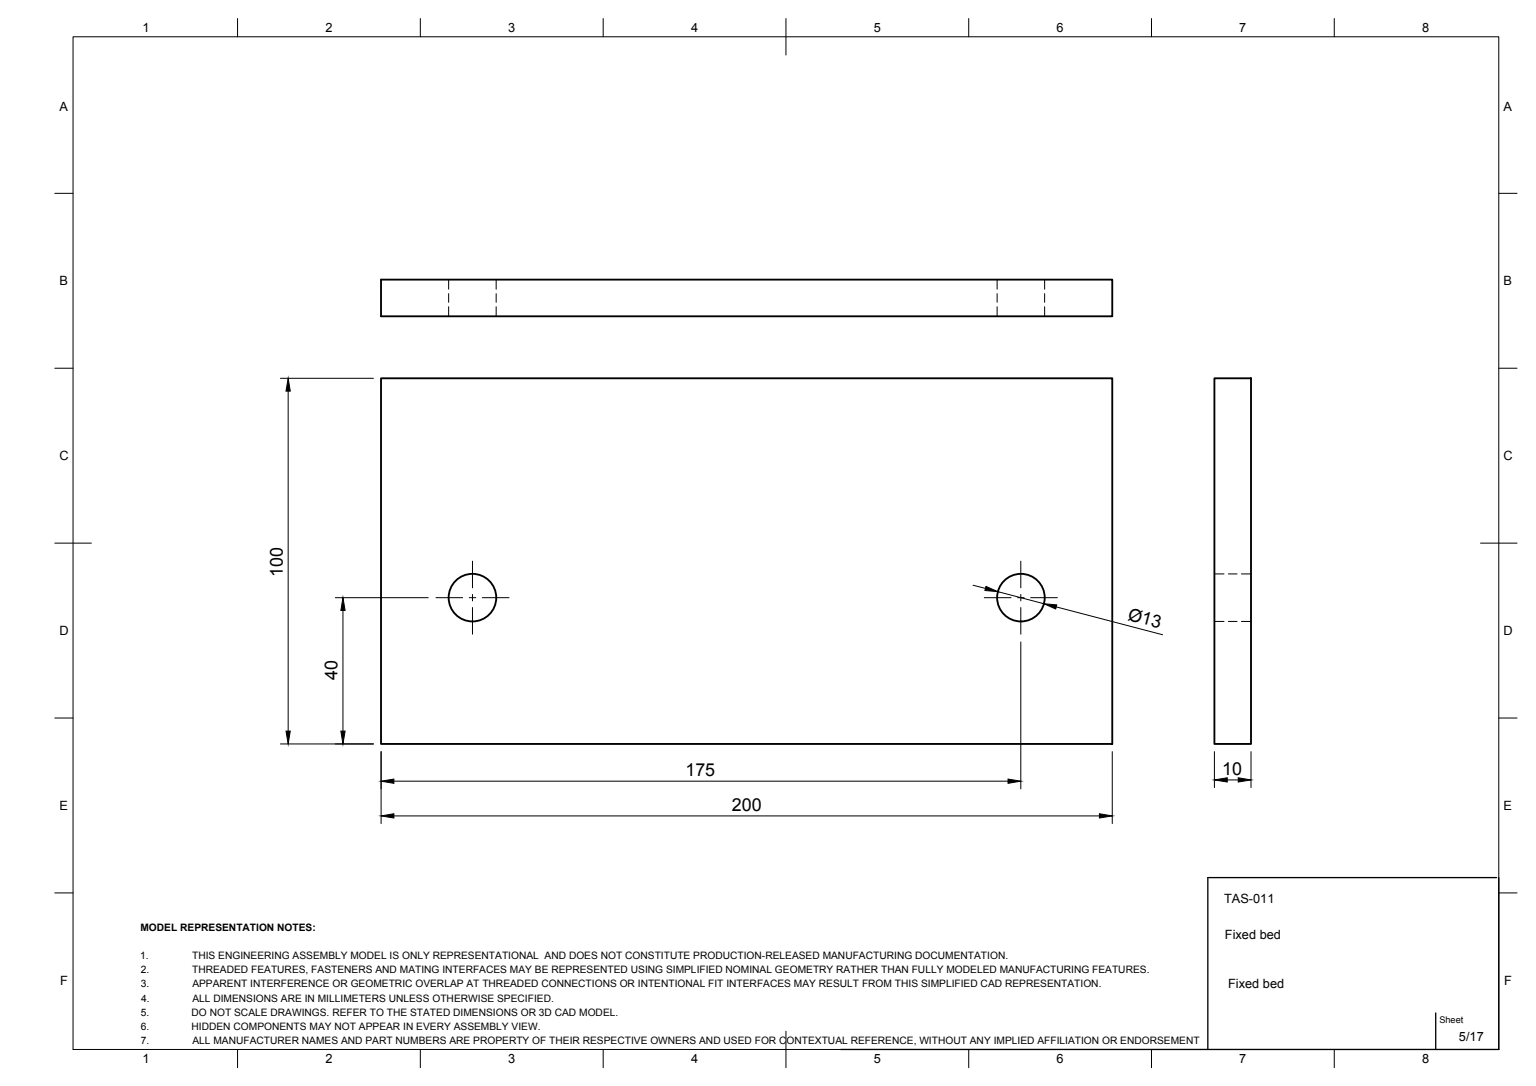
ISO-10303-21;
HEADER;
/* Generated by software containing ST-Developer
 * from STEP Tools, Inc. (www.steptools.com) 
 */

FILE_DESCRIPTION(
/* description */ (
'Independent manual bench leaf bending machine,200mm work width. Fabri
cated welded frame and folding leaf, repeated bushed and fully retaine
d hinge hardware, two handles with bonded grips, beveled clamping beam
 and modeledM12 clamp screws.2mm omitted-workpiece assembly reference 
gap, not a capacity claim. Native135deg hinge travel. Weld sizing, pro
duction fits, material condition, bending capacity, strength and life 
unassigned.'),
/* implementation_level */ '2;1');

FILE_NAME(
/* name */ 'Fixed bed.step',
/* time_stamp */ '2026-11-14T09:11:34-08:00',
/* author */ (''),
/* organization */ (''),
/* preprocessor_version */ 'ST-DEVELOPER v20.2',
/* originating_system */ 'Autodesk Translation Framework v15.17.0.0',
/* authorisation */ '');

FILE_SCHEMA (('AUTOMOTIVE_DESIGN { 1 0 10303 214 3 1 1 }'));
ENDSEC;

DATA;
#10=MECHANICAL_DESIGN_GEOMETRIC_PRESENTATION_REPRESENTATION('',(#447),#37701);
#411=SHAPE_REPRESENTATION_RELATIONSHIP('SRR','None',#37780,#429);
#429=ADVANCED_BREP_SHAPE_REPRESENTATION('',(#465),#37684);
#447=STYLED_ITEM('',(#37879),#465);
#465=MANIFOLD_SOLID_BREP('Body1',#4145);
#490=FACE_BOUND('',#843,.T.);
#491=FACE_BOUND('',#844,.T.);
#492=FACE_BOUND('',#846,.T.);
#493=FACE_BOUND('',#847,.T.);
#522=PLANE('',#4400);
#523=PLANE('',#4401);
#524=PLANE('',#4402);
#525=PLANE('',#4403);
#526=PLANE('',#4404);
#527=PLANE('',#4405);
#616=FACE_OUTER_BOUND('',#836,.T.);
#617=FACE_OUTER_BOUND('',#837,.T.);
#618=FACE_OUTER_BOUND('',#838,.T.);
#619=FACE_OUTER_BOUND('',#839,.T.);
#620=FACE_OUTER_BOUND('',#840,.T.);
#621=FACE_OUTER_BOUND('',#841,.T.);
#622=FACE_OUTER_BOUND('',#842,.T.);
#623=FACE_OUTER_BOUND('',#845,.T.);
#836=EDGE_LOOP('',(#2711,#2712,#2713,#2714));
#837=EDGE_LOOP('',(#2715,#2716,#2717,#2718));
#838=EDGE_LOOP('',(#2719,#2720,#2721,#2722));
#839=EDGE_LOOP('',(#2723,#2724,#2725,#2726));
#840=EDGE_LOOP('',(#2727,#2728,#2729,#2730));
#841=EDGE_LOOP('',(#2731,#2732,#2733,#2734));
#842=EDGE_LOOP('',(#2735,#2736,#2737,#2738));
#843=EDGE_LOOP('',(#2739));
#844=EDGE_LOOP('',(#2740));
#845=EDGE_LOOP('',(#2741,#2742,#2743,#2744));
#846=EDGE_LOOP('',(#2745));
#847=EDGE_LOOP('',(#2746));
#1080=LINE('',#5729,#1329);
#1081=LINE('',#5735,#1330);
#1082=LINE('',#5740,#1331);
#1083=LINE('',#5742,#1332);
#1084=LINE('',#5744,#1333);
#1085=LINE('',#5745,#1334);
#1086=LINE('',#5748,#1335);
#1087=LINE('',#5750,#1336);
#1088=LINE('',#5751,#1337);
#1089=LINE('',#5754,#1338);
#1090=LINE('',#5756,#1339);
#1091=LINE('',#5757,#1340);
#1092=LINE('',#5759,#1341);
#1093=LINE('',#5760,#1342);
#1329=VECTOR('',#4797,6.5);
#1330=VECTOR('',#4804,6.5);
#1331=VECTOR('',#4809,10.);
#1332=VECTOR('',#4810,10.);
#1333=VECTOR('',#4811,10.);
#1334=VECTOR('',#4812,10.);
#1335=VECTOR('',#4815,10.);
#1336=VECTOR('',#4816,10.);
#1337=VECTOR('',#4817,10.);
#1338=VECTOR('',#4820,10.);
#1339=VECTOR('',#4821,10.);
#1340=VECTOR('',#4822,10.);
#1341=VECTOR('',#4825,10.);
#1342=VECTOR('',#4826,10.);
#1574=CIRCLE('',#4395,6.5);
#1575=CIRCLE('',#4396,6.5);
#1576=CIRCLE('',#4398,6.5);
#1577=CIRCLE('',#4399,6.5);
#1661=VERTEX_POINT('',#5726);
#1662=VERTEX_POINT('',#5728);
#1663=VERTEX_POINT('',#5732);
#1664=VERTEX_POINT('',#5734);
#1665=VERTEX_POINT('',#5738);
#1666=VERTEX_POINT('',#5739);
#1667=VERTEX_POINT('',#5741);
#1668=VERTEX_POINT('',#5743);
#1669=VERTEX_POINT('',#5747);
#1670=VERTEX_POINT('',#5749);
#1671=VERTEX_POINT('',#5753);
#1672=VERTEX_POINT('',#5755);
#2089=EDGE_CURVE('',#1661,#1661,#1574,.T.);
#2090=EDGE_CURVE('',#1661,#1662,#1080,.T.);
#2091=EDGE_CURVE('',#1662,#1662,#1575,.T.);
#2092=EDGE_CURVE('',#1663,#1663,#1576,.T.);
#2093=EDGE_CURVE('',#1663,#1664,#1081,.T.);
#2094=EDGE_CURVE('',#1664,#1664,#1577,.T.);
#2095=EDGE_CURVE('',#1665,#1666,#1082,.T.);
#2096=EDGE_CURVE('',#1666,#1667,#1083,.T.);
#2097=EDGE_CURVE('',#1668,#1667,#1084,.T.);
#2098=EDGE_CURVE('',#1665,#1668,#1085,.T.);
#2099=EDGE_CURVE('',#1669,#1665,#1086,.T.);
#2100=EDGE_CURVE('',#1670,#1668,#1087,.T.);
#2101=EDGE_CURVE('',#1669,#1670,#1088,.T.);
#2102=EDGE_CURVE('',#1671,#1669,#1089,.T.);
#2103=EDGE_CURVE('',#1672,#1670,#1090,.T.);
#2104=EDGE_CURVE('',#1671,#1672,#1091,.T.);
#2105=EDGE_CURVE('',#1666,#1671,#1092,.T.);
#2106=EDGE_CURVE('',#1667,#1672,#1093,.T.);
#2711=ORIENTED_EDGE('',*,*,#2089,.F.);
#2712=ORIENTED_EDGE('',*,*,#2090,.T.);
#2713=ORIENTED_EDGE('',*,*,#2091,.F.);
#2714=ORIENTED_EDGE('',*,*,#2090,.F.);
#2715=ORIENTED_EDGE('',*,*,#2092,.F.);
#2716=ORIENTED_EDGE('',*,*,#2093,.T.);
#2717=ORIENTED_EDGE('',*,*,#2094,.F.);
#2718=ORIENTED_EDGE('',*,*,#2093,.F.);
#2719=ORIENTED_EDGE('',*,*,#2095,.T.);
#2720=ORIENTED_EDGE('',*,*,#2096,.T.);
#2721=ORIENTED_EDGE('',*,*,#2097,.F.);
#2722=ORIENTED_EDGE('',*,*,#2098,.F.);
#2723=ORIENTED_EDGE('',*,*,#2099,.T.);
#2724=ORIENTED_EDGE('',*,*,#2098,.T.);
#2725=ORIENTED_EDGE('',*,*,#2100,.F.);
#2726=ORIENTED_EDGE('',*,*,#2101,.F.);
#2727=ORIENTED_EDGE('',*,*,#2102,.T.);
#2728=ORIENTED_EDGE('',*,*,#2101,.T.);
#2729=ORIENTED_EDGE('',*,*,#2103,.F.);
#2730=ORIENTED_EDGE('',*,*,#2104,.F.);
#2731=ORIENTED_EDGE('',*,*,#2105,.T.);
#2732=ORIENTED_EDGE('',*,*,#2104,.T.);
#2733=ORIENTED_EDGE('',*,*,#2106,.F.);
#2734=ORIENTED_EDGE('',*,*,#2096,.F.);
#2735=ORIENTED_EDGE('',*,*,#2106,.T.);
#2736=ORIENTED_EDGE('',*,*,#2103,.T.);
#2737=ORIENTED_EDGE('',*,*,#2100,.T.);
#2738=ORIENTED_EDGE('',*,*,#2097,.T.);
#2739=ORIENTED_EDGE('',*,*,#2089,.T.);
#2740=ORIENTED_EDGE('',*,*,#2092,.T.);
#2741=ORIENTED_EDGE('',*,*,#2105,.F.);
#2742=ORIENTED_EDGE('',*,*,#2095,.F.);
#2743=ORIENTED_EDGE('',*,*,#2099,.F.);
#2744=ORIENTED_EDGE('',*,*,#2102,.F.);
#2745=ORIENTED_EDGE('',*,*,#2091,.T.);
#2746=ORIENTED_EDGE('',*,*,#2094,.T.);
#3819=CYLINDRICAL_SURFACE('',#4394,6.5);
#3820=CYLINDRICAL_SURFACE('',#4397,6.5);
#3946=ADVANCED_FACE('',(#616),#3819,.F.);
#3947=ADVANCED_FACE('',(#617),#3820,.F.);
#3948=ADVANCED_FACE('',(#618),#522,.T.);
#3949=ADVANCED_FACE('',(#619),#523,.T.);
#3950=ADVANCED_FACE('',(#620),#524,.T.);
#3951=ADVANCED_FACE('',(#621),#525,.T.);
#3952=ADVANCED_FACE('',(#622,#490,#491),#526,.T.);
#3953=ADVANCED_FACE('',(#623,#492,#493),#527,.F.);
#4145=CLOSED_SHELL('',(#3946,#3947,#3948,#3949,#3950,#3951,#3952,#3953));
#4393=AXIS2_PLACEMENT_3D('',#5724,#4791,#4792);
#4394=AXIS2_PLACEMENT_3D('',#5725,#4793,#4794);
#4395=AXIS2_PLACEMENT_3D('',#5727,#4795,#4796);
#4396=AXIS2_PLACEMENT_3D('',#5730,#4798,#4799);
#4397=AXIS2_PLACEMENT_3D('',#5731,#4800,#4801);
#4398=AXIS2_PLACEMENT_3D('',#5733,#4802,#4803);
#4399=AXIS2_PLACEMENT_3D('',#5736,#4805,#4806);
#4400=AXIS2_PLACEMENT_3D('',#5737,#4807,#4808);
#4401=AXIS2_PLACEMENT_3D('',#5746,#4813,#4814);
#4402=AXIS2_PLACEMENT_3D('',#5752,#4818,#4819);
#4403=AXIS2_PLACEMENT_3D('',#5758,#4823,#4824);
#4404=AXIS2_PLACEMENT_3D('',#5761,#4827,#4828);
#4405=AXIS2_PLACEMENT_3D('',#5762,#4829,#4830);
#4791=DIRECTION('axis',(0.,0.,1.));
#4792=DIRECTION('refdir',(1.,0.,0.));
#4793=DIRECTION('center_axis',(0.,0.,-1.));
#4794=DIRECTION('ref_axis',(1.,0.,0.));
#4795=DIRECTION('center_axis',(0.,0.,-1.));
#4796=DIRECTION('ref_axis',(1.,0.,0.));
#4797=DIRECTION('',(0.,0.,-1.));
#4798=DIRECTION('center_axis',(0.,0.,1.));
#4799=DIRECTION('ref_axis',(1.,0.,0.));
#4800=DIRECTION('center_axis',(0.,0.,-1.));
#4801=DIRECTION('ref_axis',(1.,0.,0.));
#4802=DIRECTION('center_axis',(0.,0.,-1.));
#4803=DIRECTION('ref_axis',(1.,0.,0.));
#4804=DIRECTION('',(0.,0.,-1.));
#4805=DIRECTION('center_axis',(0.,0.,1.));
#4806=DIRECTION('ref_axis',(1.,0.,0.));
#4807=DIRECTION('center_axis',(0.,1.,0.));
#4808=DIRECTION('ref_axis',(-1.,0.,0.));
#4809=DIRECTION('',(-1.,0.,0.));
#4810=DIRECTION('',(0.,0.,1.));
#4811=DIRECTION('',(-1.,0.,0.));
#4812=DIRECTION('',(0.,0.,1.));
#4813=DIRECTION('center_axis',(1.,0.,0.));
#4814=DIRECTION('ref_axis',(0.,1.,0.));
#4815=DIRECTION('',(0.,1.,0.));
#4816=DIRECTION('',(0.,1.,0.));
#4817=DIRECTION('',(0.,0.,1.));
#4818=DIRECTION('center_axis',(0.,-1.,0.));
#4819=DIRECTION('ref_axis',(1.,0.,0.));
#4820=DIRECTION('',(1.,0.,0.));
#4821=DIRECTION('',(1.,0.,0.));
#4822=DIRECTION('',(0.,0.,1.));
#4823=DIRECTION('center_axis',(-1.,0.,0.));
#4824=DIRECTION('ref_axis',(0.,-1.,0.));
#4825=DIRECTION('',(0.,-1.,0.));
#4826=DIRECTION('',(0.,-1.,0.));
#4827=DIRECTION('center_axis',(0.,0.,1.));
#4828=DIRECTION('ref_axis',(1.,0.,0.));
#4829=DIRECTION('center_axis',(0.,0.,1.));
#4830=DIRECTION('ref_axis',(1.,0.,0.));
#5724=CARTESIAN_POINT('',(0.,0.,0.));
#5725=CARTESIAN_POINT('Origin',(-60.,-75.,35.));
#5726=CARTESIAN_POINT('',(-66.5,-75.,40.));
#5727=CARTESIAN_POINT('Origin',(-60.,-75.,40.));
#5728=CARTESIAN_POINT('',(-66.5,-75.,30.));
#5729=CARTESIAN_POINT('',(-66.5,-75.,35.));
#5730=CARTESIAN_POINT('Origin',(-60.,-75.,30.));
#5731=CARTESIAN_POINT('Origin',(-60.,75.,35.));
#5732=CARTESIAN_POINT('',(-66.5,75.,40.));
#5733=CARTESIAN_POINT('Origin',(-60.,75.,40.));
#5734=CARTESIAN_POINT('',(-66.5,75.,30.));
#5735=CARTESIAN_POINT('',(-66.5,75.,35.));
#5736=CARTESIAN_POINT('Origin',(-60.,75.,30.));
#5737=CARTESIAN_POINT('Origin',(0.,100.,30.));
#5738=CARTESIAN_POINT('',(0.,100.,30.));
#5739=CARTESIAN_POINT('',(-100.,100.,30.));
#5740=CARTESIAN_POINT('',(0.,100.,30.));
#5741=CARTESIAN_POINT('',(-100.,100.,40.));
#5742=CARTESIAN_POINT('',(-100.,100.,30.));
#5743=CARTESIAN_POINT('',(0.,100.,40.));
#5744=CARTESIAN_POINT('',(0.,100.,40.));
#5745=CARTESIAN_POINT('',(0.,100.,30.));
#5746=CARTESIAN_POINT('Origin',(0.,-100.,30.));
#5747=CARTESIAN_POINT('',(0.,-100.,30.));
#5748=CARTESIAN_POINT('',(0.,-100.,30.));
#5749=CARTESIAN_POINT('',(0.,-100.,40.));
#5750=CARTESIAN_POINT('',(0.,-100.,40.));
#5751=CARTESIAN_POINT('',(0.,-100.,30.));
#5752=CARTESIAN_POINT('Origin',(-100.,-100.,30.));
#5753=CARTESIAN_POINT('',(-100.,-100.,30.));
#5754=CARTESIAN_POINT('',(-100.,-100.,30.));
#5755=CARTESIAN_POINT('',(-100.,-100.,40.));
#5756=CARTESIAN_POINT('',(-100.,-100.,40.));
#5757=CARTESIAN_POINT('',(-100.,-100.,30.));
#5758=CARTESIAN_POINT('Origin',(-100.,100.,30.));
#5759=CARTESIAN_POINT('',(-100.,100.,30.));
#5760=CARTESIAN_POINT('',(-100.,100.,40.));
#5761=CARTESIAN_POINT('Origin',(-50.,0.,40.));
#5762=CARTESIAN_POINT('Origin',(-50.,0.,30.));
#37664=UNCERTAINTY_MEASURE_WITH_UNIT(LENGTH_MEASURE(0.01),#37702,
'DISTANCE_ACCURACY_VALUE',
'Maximum model space distance between geometric entities at asserted c
onnectivities');
#37681=UNCERTAINTY_MEASURE_WITH_UNIT(LENGTH_MEASURE(0.01),#37702,
'DISTANCE_ACCURACY_VALUE',
'Maximum model space distance between geometric entities at asserted c
onnectivities');
#37684=(
GEOMETRIC_REPRESENTATION_CONTEXT(3)
GLOBAL_UNCERTAINTY_ASSIGNED_CONTEXT((#37664))
GLOBAL_UNIT_ASSIGNED_CONTEXT((#37702,#37704,#37705))
REPRESENTATION_CONTEXT('','3D')
);
#37701=(
GEOMETRIC_REPRESENTATION_CONTEXT(3)
GLOBAL_UNCERTAINTY_ASSIGNED_CONTEXT((#37681))
GLOBAL_UNIT_ASSIGNED_CONTEXT((#37702,#37704,#37705))
REPRESENTATION_CONTEXT('','3D')
);
#37702=(
LENGTH_UNIT()
NAMED_UNIT(*)
SI_UNIT(.MILLI.,.METRE.)
);
#37704=(
NAMED_UNIT(*)
PLANE_ANGLE_UNIT()
SI_UNIT($,.RADIAN.)
);
#37705=(
NAMED_UNIT(*)
SI_UNIT($,.STERADIAN.)
SOLID_ANGLE_UNIT()
);
#37708=SHAPE_DEFINITION_REPRESENTATION(#37727,#37780);
#37727=PRODUCT_DEFINITION_SHAPE('',$,#37800);
#37780=SHAPE_REPRESENTATION('',(#4393),#37684);
#37797=PRODUCT_DEFINITION_CONTEXT('part definition',#37856,'design');
#37800=PRODUCT_DEFINITION('Fixed bed','Fixed bed',#37819,#37797);
#37819=PRODUCT_DEFINITION_FORMATION('',$,#37860);
#37856=APPLICATION_CONTEXT(
'Core Data for Automotive Mechanical Design Process');
#37857=PRODUCT_CONTEXT('part definition',#37856,'mechanical');
#37860=PRODUCT('Fixed bed','Fixed bed',$,(#37857));
#37879=PRESENTATION_STYLE_ASSIGNMENT((#37887));
#37887=SURFACE_STYLE_USAGE(.BOTH.,#37895);
#37895=SURFACE_SIDE_STYLE('',(#37903));
#37903=SURFACE_STYLE_FILL_AREA(#37911);
#37911=FILL_AREA_STYLE('Opaque(104,114,127)',(#37919));
#37919=FILL_AREA_STYLE_COLOUR('Opaque(104,114,127)',#37927);
#37927=COLOUR_RGB('Opaque(104,114,127)',0.407843137254902,0.447058823529412,
0.498039215686275);
ENDSEC;
END-ISO-10303-21;
